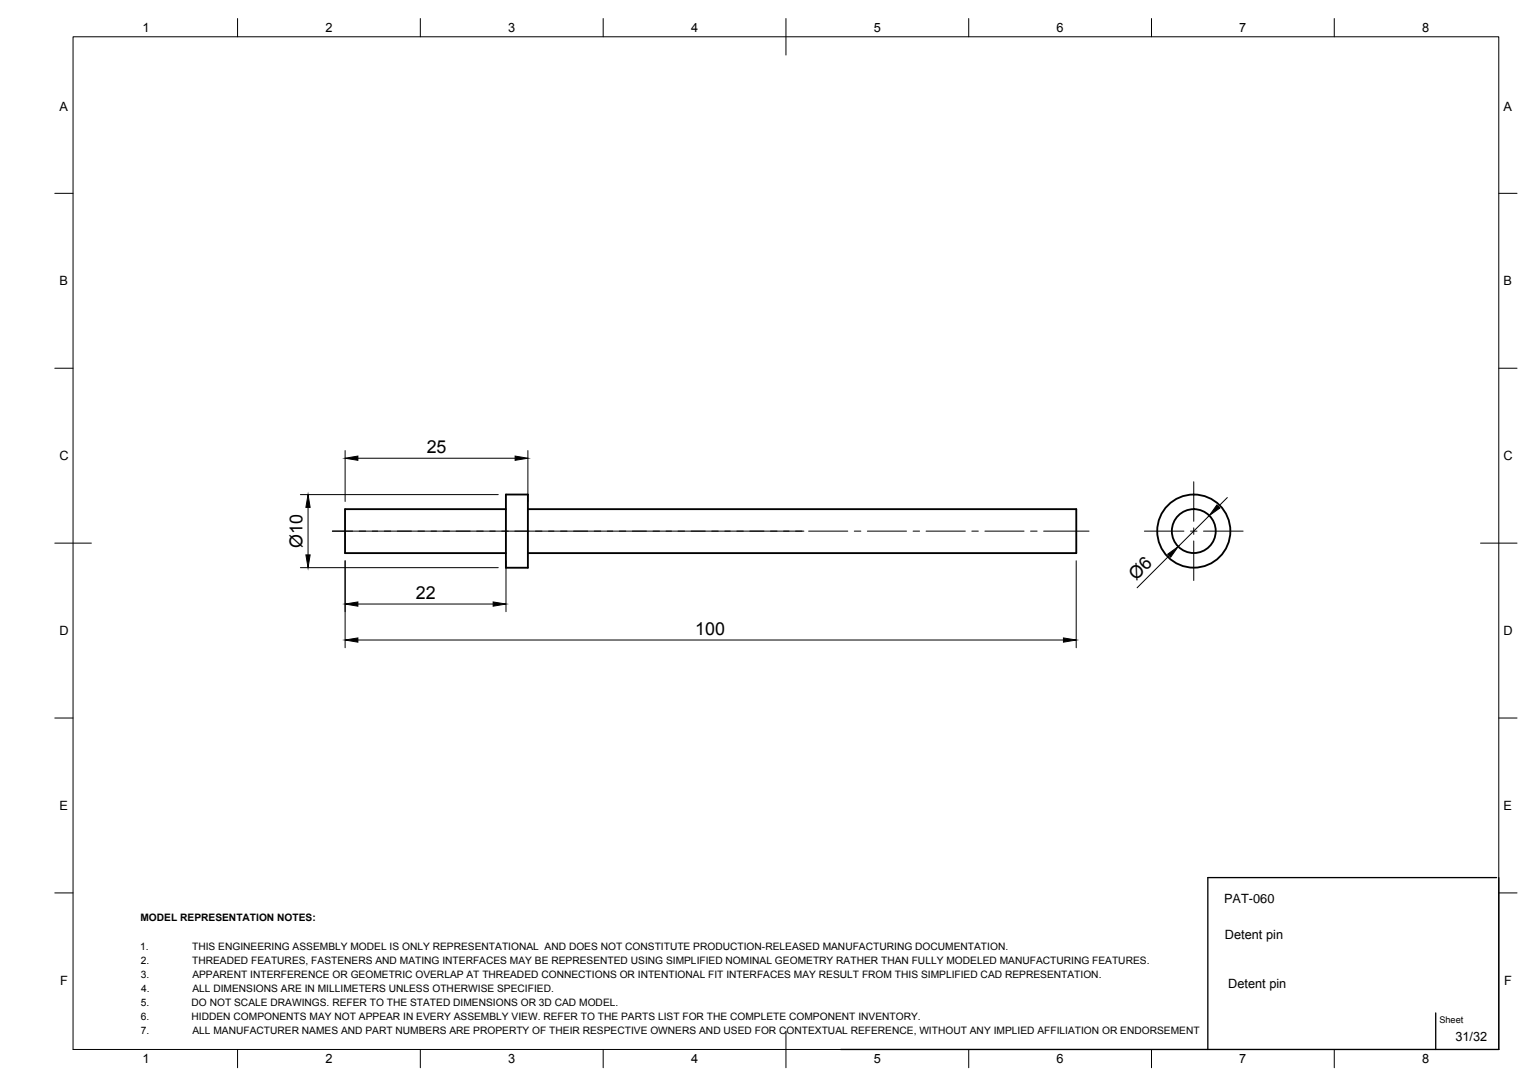
ISO-10303-21;
HEADER;
/* Generated by software containing ST-Developer
 * from STEP Tools, Inc. (www.steptools.com) 
 */

FILE_DESCRIPTION(
/* description */ ('Indexing fixture plate with plunger'),
/* implementation_level */ '2;1');

FILE_NAME(
/* name */ 'Detent pin.step',
/* time_stamp */ '2026-10-28T03:23:41-07:00',
/* author */ (''),
/* organization */ (''),
/* preprocessor_version */ 'ST-DEVELOPER v20.2',
/* originating_system */ 'Autodesk Translation Framework v15.17.0.0',
/* authorisation */ '');

FILE_SCHEMA (('AUTOMOTIVE_DESIGN { 1 0 10303 214 3 1 1 }'));
ENDSEC;

DATA;
#10=MECHANICAL_DESIGN_GEOMETRIC_PRESENTATION_REPRESENTATION('',(#350),#10020);
#287=SHAPE_REPRESENTATION_RELATIONSHIP('SRR','None',#10164,#314);
#314=ADVANCED_BREP_SHAPE_REPRESENTATION('',(#384),#10017);
#350=STYLED_ITEM('',(#10368),#384);
#384=MANIFOLD_SOLID_BREP('Body1',#4606);
#530=FACE_BOUND('',#1361,.T.);
#531=FACE_BOUND('',#1363,.T.);
#653=PLANE('',#5523);
#654=PLANE('',#5525);
#655=PLANE('',#5528);
#656=PLANE('',#5535);
#930=FACE_OUTER_BOUND('',#1359,.T.);
#931=FACE_OUTER_BOUND('',#1360,.T.);
#932=FACE_OUTER_BOUND('',#1362,.T.);
#933=FACE_OUTER_BOUND('',#1364,.T.);
#934=FACE_OUTER_BOUND('',#1365,.T.);
#935=FACE_OUTER_BOUND('',#1366,.T.);
#936=FACE_OUTER_BOUND('',#1367,.T.);
#1359=EDGE_LOOP('',(#4067));
#1360=EDGE_LOOP('',(#4068));
#1361=EDGE_LOOP('',(#4069));
#1362=EDGE_LOOP('',(#4070));
#1363=EDGE_LOOP('',(#4071));
#1364=EDGE_LOOP('',(#4072,#4073,#4074,#4075));
#1365=EDGE_LOOP('',(#4076,#4077,#4078,#4079));
#1366=EDGE_LOOP('',(#4080,#4081,#4082,#4083));
#1367=EDGE_LOOP('',(#4084));
#1583=LINE('',#9807,#1803);
#1584=LINE('',#9809,#1804);
#1585=LINE('',#9813,#1805);
#1803=VECTOR('',#7014,0.5);
#1804=VECTOR('',#7017,0.3);
#1805=VECTOR('',#7022,0.3);
#2119=CIRCLE('',#5524,0.3);
#2120=CIRCLE('',#5526,0.5);
#2121=CIRCLE('',#5527,0.3);
#2122=CIRCLE('',#5529,0.5);
#2123=CIRCLE('',#5530,0.3);
#2124=CIRCLE('',#5534,0.3);
#2478=VERTEX_POINT('',#9794);
#2479=VERTEX_POINT('',#9797);
#2480=VERTEX_POINT('',#9799);
#2481=VERTEX_POINT('',#9802);
#2482=VERTEX_POINT('',#9804);
#2483=VERTEX_POINT('',#9811);
#3013=EDGE_CURVE('',#2478,#2478,#2119,.T.);
#3014=EDGE_CURVE('',#2479,#2479,#2120,.T.);
#3015=EDGE_CURVE('',#2480,#2480,#2121,.T.);
#3016=EDGE_CURVE('',#2481,#2481,#2122,.T.);
#3017=EDGE_CURVE('',#2482,#2482,#2123,.T.);
#3018=EDGE_CURVE('',#2479,#2481,#1583,.T.);
#3019=EDGE_CURVE('',#2482,#2478,#1584,.T.);
#3020=EDGE_CURVE('',#2483,#2483,#2124,.T.);
#3021=EDGE_CURVE('',#2483,#2480,#1585,.T.);
#4067=ORIENTED_EDGE('',*,*,#3013,.F.);
#4068=ORIENTED_EDGE('',*,*,#3014,.T.);
#4069=ORIENTED_EDGE('',*,*,#3015,.F.);
#4070=ORIENTED_EDGE('',*,*,#3016,.F.);
#4071=ORIENTED_EDGE('',*,*,#3017,.F.);
#4072=ORIENTED_EDGE('',*,*,#3014,.F.);
#4073=ORIENTED_EDGE('',*,*,#3018,.T.);
#4074=ORIENTED_EDGE('',*,*,#3016,.T.);
#4075=ORIENTED_EDGE('',*,*,#3018,.F.);
#4076=ORIENTED_EDGE('',*,*,#3017,.T.);
#4077=ORIENTED_EDGE('',*,*,#3019,.T.);
#4078=ORIENTED_EDGE('',*,*,#3013,.T.);
#4079=ORIENTED_EDGE('',*,*,#3019,.F.);
#4080=ORIENTED_EDGE('',*,*,#3020,.F.);
#4081=ORIENTED_EDGE('',*,*,#3021,.T.);
#4082=ORIENTED_EDGE('',*,*,#3015,.T.);
#4083=ORIENTED_EDGE('',*,*,#3021,.F.);
#4084=ORIENTED_EDGE('',*,*,#3020,.T.);
#4278=CYLINDRICAL_SURFACE('',#5531,0.5);
#4279=CYLINDRICAL_SURFACE('',#5532,0.3);
#4280=CYLINDRICAL_SURFACE('',#5533,0.3);
#4545=ADVANCED_FACE('',(#930),#653,.F.);
#4546=ADVANCED_FACE('',(#931,#530),#654,.T.);
#4547=ADVANCED_FACE('',(#932,#531),#655,.F.);
#4548=ADVANCED_FACE('',(#933),#4278,.T.);
#4549=ADVANCED_FACE('',(#934),#4279,.T.);
#4550=ADVANCED_FACE('',(#935),#4280,.T.);
#4551=ADVANCED_FACE('',(#936),#656,.T.);
#4606=CLOSED_SHELL('',(#4545,#4546,#4547,#4548,#4549,#4550,#4551));
#5522=AXIS2_PLACEMENT_3D('',#9792,#6994,#6995);
#5523=AXIS2_PLACEMENT_3D('',#9793,#6996,#6997);
#5524=AXIS2_PLACEMENT_3D('',#9795,#6998,#6999);
#5525=AXIS2_PLACEMENT_3D('',#9796,#7000,#7001);
#5526=AXIS2_PLACEMENT_3D('',#9798,#7002,#7003);
#5527=AXIS2_PLACEMENT_3D('',#9800,#7004,#7005);
#5528=AXIS2_PLACEMENT_3D('',#9801,#7006,#7007);
#5529=AXIS2_PLACEMENT_3D('',#9803,#7008,#7009);
#5530=AXIS2_PLACEMENT_3D('',#9805,#7010,#7011);
#5531=AXIS2_PLACEMENT_3D('',#9806,#7012,#7013);
#5532=AXIS2_PLACEMENT_3D('',#9808,#7015,#7016);
#5533=AXIS2_PLACEMENT_3D('',#9810,#7018,#7019);
#5534=AXIS2_PLACEMENT_3D('',#9812,#7020,#7021);
#5535=AXIS2_PLACEMENT_3D('',#9814,#7023,#7024);
#6994=DIRECTION('axis',(0.,0.,1.));
#6995=DIRECTION('refdir',(1.,0.,0.));
#6996=DIRECTION('center_axis',(0.,0.,1.));
#6997=DIRECTION('ref_axis',(1.,0.,0.));
#6998=DIRECTION('center_axis',(0.,0.,1.));
#6999=DIRECTION('ref_axis',(1.,0.,0.));
#7000=DIRECTION('center_axis',(0.,0.,1.));
#7001=DIRECTION('ref_axis',(1.,0.,0.));
#7002=DIRECTION('center_axis',(0.,0.,1.));
#7003=DIRECTION('ref_axis',(1.,0.,0.));
#7004=DIRECTION('center_axis',(0.,0.,1.));
#7005=DIRECTION('ref_axis',(1.,0.,0.));
#7006=DIRECTION('center_axis',(0.,0.,1.));
#7007=DIRECTION('ref_axis',(1.,0.,0.));
#7008=DIRECTION('center_axis',(0.,0.,1.));
#7009=DIRECTION('ref_axis',(1.,0.,0.));
#7010=DIRECTION('center_axis',(0.,0.,-1.));
#7011=DIRECTION('ref_axis',(1.,0.,0.));
#7012=DIRECTION('center_axis',(0.,0.,1.));
#7013=DIRECTION('ref_axis',(1.,0.,0.));
#7014=DIRECTION('',(0.,0.,-1.));
#7015=DIRECTION('center_axis',(0.,0.,1.));
#7016=DIRECTION('ref_axis',(1.,0.,0.));
#7017=DIRECTION('',(0.,0.,-1.));
#7018=DIRECTION('center_axis',(0.,0.,1.));
#7019=DIRECTION('ref_axis',(1.,0.,0.));
#7020=DIRECTION('center_axis',(0.,0.,1.));
#7021=DIRECTION('ref_axis',(1.,0.,0.));
#7022=DIRECTION('',(0.,0.,-1.));
#7023=DIRECTION('center_axis',(0.,0.,1.));
#7024=DIRECTION('ref_axis',(1.,0.,0.));
#9792=CARTESIAN_POINT('',(0.,0.,0.));
#9793=CARTESIAN_POINT('Origin',(7.2,0.,-3.));
#9794=CARTESIAN_POINT('',(6.9,-3.67394039744206E-17,-3.));
#9795=CARTESIAN_POINT('Origin',(7.2,0.,-3.));
#9796=CARTESIAN_POINT('Origin',(7.2,0.,4.8));
#9797=CARTESIAN_POINT('',(6.7,-6.12323399573677E-17,4.8));
#9798=CARTESIAN_POINT('Origin',(7.2,0.,4.8));
#9799=CARTESIAN_POINT('',(6.9,-3.67394039744206E-17,4.8));
#9800=CARTESIAN_POINT('Origin',(7.2,0.,4.8));
#9801=CARTESIAN_POINT('Origin',(7.2,0.,4.5));
#9802=CARTESIAN_POINT('',(6.7,-6.12323399573677E-17,4.5));
#9803=CARTESIAN_POINT('Origin',(7.2,0.,4.5));
#9804=CARTESIAN_POINT('',(6.9,3.67394039744206E-17,4.5));
#9805=CARTESIAN_POINT('Origin',(7.2,0.,4.5));
#9806=CARTESIAN_POINT('Origin',(7.2,0.,4.5));
#9807=CARTESIAN_POINT('',(6.7,-6.12323399573677E-17,4.5));
#9808=CARTESIAN_POINT('Origin',(7.2,0.,-1.5));
#9809=CARTESIAN_POINT('',(6.9,-3.67394039744206E-17,-1.5));
#9810=CARTESIAN_POINT('Origin',(7.2,0.,-1.5));
#9811=CARTESIAN_POINT('',(6.9,-3.67394039744206E-17,7.));
#9812=CARTESIAN_POINT('Origin',(7.2,0.,7.));
#9813=CARTESIAN_POINT('',(6.9,-3.67394039744206E-17,-1.5));
#9814=CARTESIAN_POINT('Origin',(7.2,0.,7.));
#9984=UNCERTAINTY_MEASURE_WITH_UNIT(LENGTH_MEASURE(0.001),#10021,
'DISTANCE_ACCURACY_VALUE',
'Maximum model space distance between geometric entities at asserted c
onnectivities');
#9987=UNCERTAINTY_MEASURE_WITH_UNIT(LENGTH_MEASURE(0.001),#10021,
'DISTANCE_ACCURACY_VALUE',
'Maximum model space distance between geometric entities at asserted c
onnectivities');
#10017=(
GEOMETRIC_REPRESENTATION_CONTEXT(3)
GLOBAL_UNCERTAINTY_ASSIGNED_CONTEXT((#9984))
GLOBAL_UNIT_ASSIGNED_CONTEXT((#10021,#10023,#10024))
REPRESENTATION_CONTEXT('','3D')
);
#10020=(
GEOMETRIC_REPRESENTATION_CONTEXT(3)
GLOBAL_UNCERTAINTY_ASSIGNED_CONTEXT((#9987))
GLOBAL_UNIT_ASSIGNED_CONTEXT((#10021,#10023,#10024))
REPRESENTATION_CONTEXT('','3D')
);
#10021=(
LENGTH_UNIT()
NAMED_UNIT(*)
SI_UNIT(.CENTI.,.METRE.)
);
#10023=(
NAMED_UNIT(*)
PLANE_ANGLE_UNIT()
SI_UNIT($,.RADIAN.)
);
#10024=(
NAMED_UNIT(*)
SI_UNIT($,.STERADIAN.)
SOLID_ANGLE_UNIT()
);
#10054=SHAPE_DEFINITION_REPRESENTATION(#10126,#10164);
#10126=PRODUCT_DEFINITION_SHAPE('',$,#10197);
#10164=SHAPE_REPRESENTATION('',(#5522),#10017);
#10167=PRODUCT_DEFINITION_CONTEXT('part definition',#10265,'design');
#10197=PRODUCT_DEFINITION('Detent pin','Detent pin',#10229,#10167);
#10229=PRODUCT_DEFINITION_FORMATION('',$,#10296);
#10265=APPLICATION_CONTEXT(
'Core Data for Automotive Mechanical Design Process');
#10266=PRODUCT_CONTEXT('part definition',#10265,'mechanical');
#10296=PRODUCT('Detent pin','Detent pin','Detent pin',(#10266));
#10362=COLOUR_RGB('Grey',0.48,0.52,0.57);
#10363=FILL_AREA_STYLE_COLOUR('',#10362);
#10364=FILL_AREA_STYLE('',(#10363));
#10365=SURFACE_STYLE_FILL_AREA(#10364);
#10366=SURFACE_SIDE_STYLE('',(#10365));
#10367=SURFACE_STYLE_USAGE(.BOTH.,#10366);
#10368=PRESENTATION_STYLE_ASSIGNMENT((#10367));
ENDSEC;
END-ISO-10303-21;
